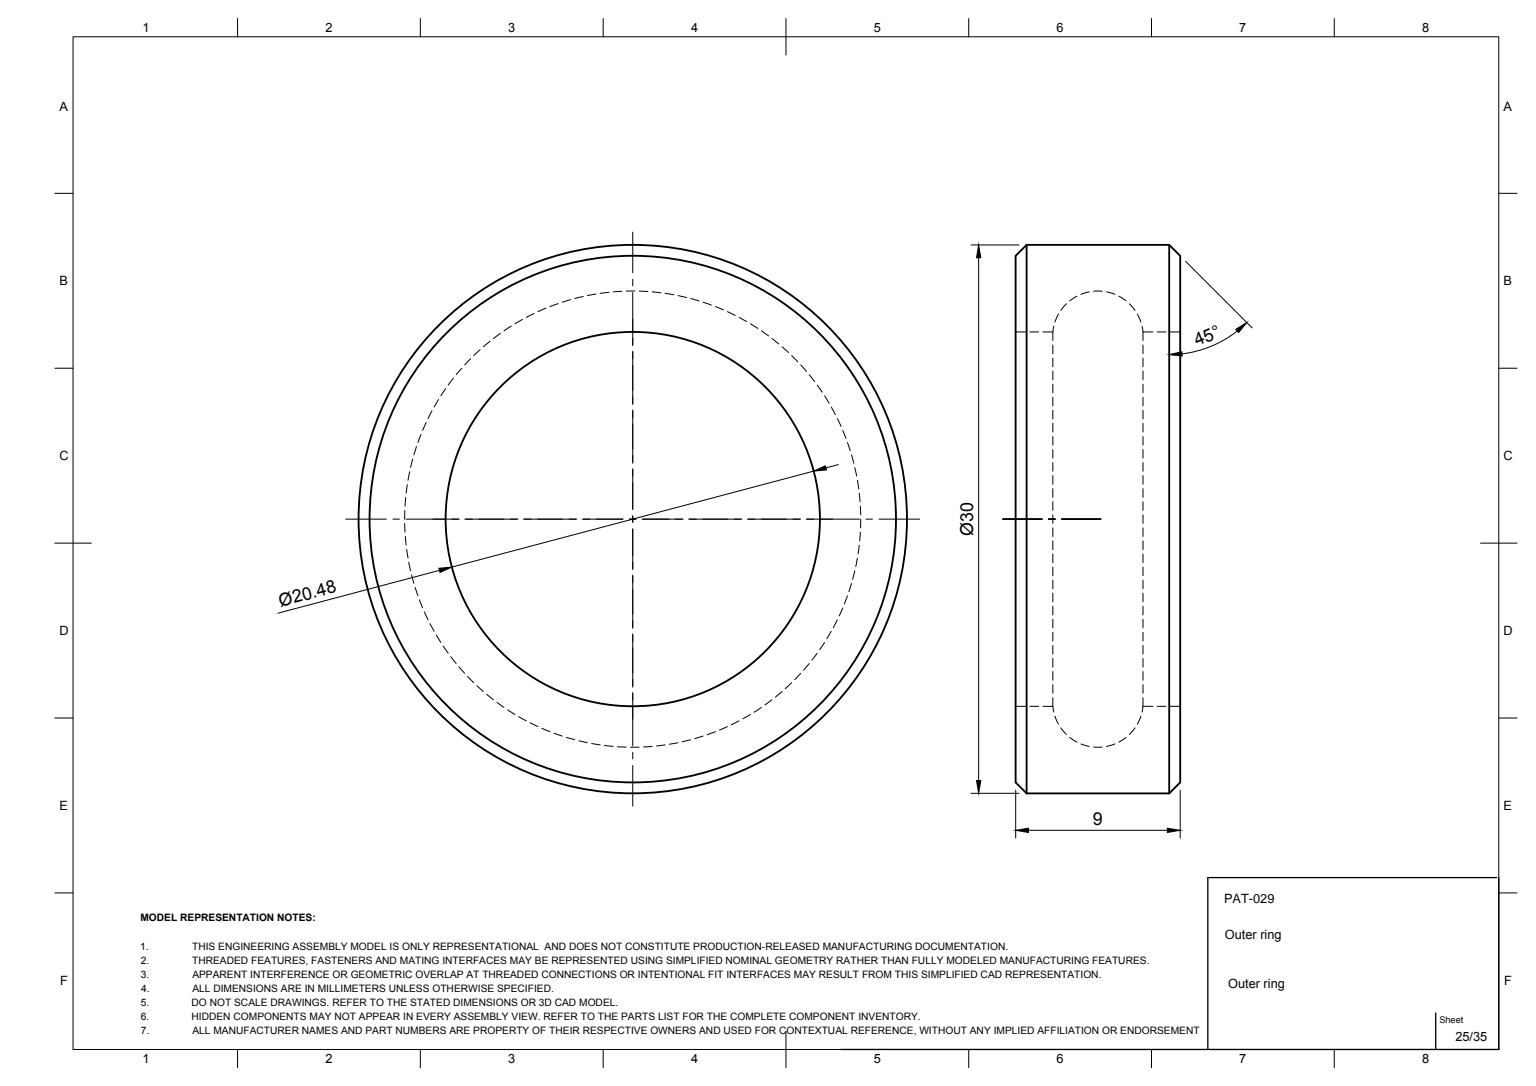
ISO-10303-21;
HEADER;
/* Generated by software containing ST-Developer
 * from STEP Tools, Inc. (www.steptools.com) 
 */

FILE_DESCRIPTION(
/* description */ ('Door-style hinge test fixture with detent'),
/* implementation_level */ '2;1');

FILE_NAME(
/* name */ 'Outer ring.step',
/* time_stamp */ '2026-10-28T03:24:57-07:00',
/* author */ (''),
/* organization */ (''),
/* preprocessor_version */ 'ST-DEVELOPER v20.2',
/* originating_system */ 'Autodesk Translation Framework v15.17.0.0',
/* authorisation */ '');

FILE_SCHEMA (('AUTOMOTIVE_DESIGN { 1 0 10303 214 3 1 1 }'));
ENDSEC;

DATA;
#10=MECHANICAL_DESIGN_GEOMETRIC_PRESENTATION_REPRESENTATION('',(#343),#9813);
#200=TOROIDAL_SURFACE('',#5464,1.,0.247676);
#206=CONICAL_SURFACE('',#5475,1.47,0.785398163397449);
#207=CONICAL_SURFACE('',#5479,1.47,0.785398163397449);
#280=SHAPE_REPRESENTATION_RELATIONSHIP('SRR','None',#9958,#311);
#311=ADVANCED_BREP_SHAPE_REPRESENTATION('',(#382),#9801);
#343=STYLED_ITEM('',(#10183),#382);
#382=MANIFOLD_SOLID_BREP('Body1',#4775);
#470=FACE_BOUND('',#1192,.T.);
#471=FACE_BOUND('',#1197,.T.);
#607=PLANE('',#5472);
#608=PLANE('',#5481);
#833=FACE_OUTER_BOUND('',#1189,.T.);
#834=FACE_OUTER_BOUND('',#1190,.T.);
#835=FACE_OUTER_BOUND('',#1191,.T.);
#836=FACE_OUTER_BOUND('',#1193,.T.);
#837=FACE_OUTER_BOUND('',#1194,.T.);
#838=FACE_OUTER_BOUND('',#1195,.T.);
#839=FACE_OUTER_BOUND('',#1196,.T.);
#840=FACE_OUTER_BOUND('',#1198,.T.);
#1189=EDGE_LOOP('',(#3931,#3932,#3933,#3934,#3935,#3936));
#1190=EDGE_LOOP('',(#3937,#3938,#3939,#3940,#3941));
#1191=EDGE_LOOP('',(#3942));
#1192=EDGE_LOOP('',(#3943));
#1193=EDGE_LOOP('',(#3944,#3945,#3946,#3947));
#1194=EDGE_LOOP('',(#3948,#3949,#3950,#3951));
#1195=EDGE_LOOP('',(#3952,#3953,#3954,#3955));
#1196=EDGE_LOOP('',(#3956));
#1197=EDGE_LOOP('',(#3957));
#1198=EDGE_LOOP('',(#3958,#3959,#3960,#3961,#3962));
#1562=LINE('',#8820,#1882);
#1563=LINE('',#8829,#1883);
#1564=LINE('',#8833,#1884);
#1565=LINE('',#8837,#1885);
#1566=LINE('',#8840,#1886);
#1882=VECTOR('',#6647,1.023815);
#1883=VECTOR('',#6658,1.47);
#1884=VECTOR('',#6663,1.5);
#1885=VECTOR('',#6668,1.47);
#1886=VECTOR('',#6673,1.023815);
#2107=CIRCLE('',#5465,1.023815);
#2108=CIRCLE('',#5466,1.023815);
#2109=CIRCLE('',#5467,0.247676);
#2110=CIRCLE('',#5468,1.023815);
#2111=CIRCLE('',#5469,1.023815);
#2112=CIRCLE('',#5471,1.023815);
#2113=CIRCLE('',#5473,1.44);
#2114=CIRCLE('',#5474,1.023815);
#2115=CIRCLE('',#5476,1.5);
#2116=CIRCLE('',#5478,1.5);
#2117=CIRCLE('',#5480,1.44);
#2462=VERTEX_POINT('',#8808);
#2463=VERTEX_POINT('',#8809);
#2464=VERTEX_POINT('',#8812);
#2465=VERTEX_POINT('',#8814);
#2466=VERTEX_POINT('',#8818);
#2467=VERTEX_POINT('',#8822);
#2468=VERTEX_POINT('',#8824);
#2469=VERTEX_POINT('',#8827);
#2470=VERTEX_POINT('',#8831);
#2471=VERTEX_POINT('',#8835);
#2982=EDGE_CURVE('',#2462,#2463,#2107,.T.);
#2983=EDGE_CURVE('',#2463,#2462,#2108,.T.);
#2984=EDGE_CURVE('',#2463,#2464,#2109,.T.);
#2985=EDGE_CURVE('',#2465,#2464,#2110,.T.);
#2986=EDGE_CURVE('',#2464,#2465,#2111,.T.);
#2987=EDGE_CURVE('',#2466,#2466,#2112,.T.);
#2988=EDGE_CURVE('',#2466,#2465,#1562,.T.);
#2989=EDGE_CURVE('',#2467,#2467,#2113,.T.);
#2990=EDGE_CURVE('',#2468,#2468,#2114,.T.);
#2991=EDGE_CURVE('',#2469,#2469,#2115,.T.);
#2992=EDGE_CURVE('',#2469,#2467,#1563,.T.);
#2993=EDGE_CURVE('',#2470,#2470,#2116,.T.);
#2994=EDGE_CURVE('',#2470,#2469,#1564,.T.);
#2995=EDGE_CURVE('',#2471,#2471,#2117,.T.);
#2996=EDGE_CURVE('',#2471,#2470,#1565,.T.);
#2997=EDGE_CURVE('',#2462,#2468,#1566,.T.);
#3931=ORIENTED_EDGE('',*,*,#2982,.F.);
#3932=ORIENTED_EDGE('',*,*,#2983,.F.);
#3933=ORIENTED_EDGE('',*,*,#2984,.T.);
#3934=ORIENTED_EDGE('',*,*,#2985,.F.);
#3935=ORIENTED_EDGE('',*,*,#2986,.F.);
#3936=ORIENTED_EDGE('',*,*,#2984,.F.);
#3937=ORIENTED_EDGE('',*,*,#2987,.T.);
#3938=ORIENTED_EDGE('',*,*,#2988,.T.);
#3939=ORIENTED_EDGE('',*,*,#2985,.T.);
#3940=ORIENTED_EDGE('',*,*,#2986,.T.);
#3941=ORIENTED_EDGE('',*,*,#2988,.F.);
#3942=ORIENTED_EDGE('',*,*,#2989,.F.);
#3943=ORIENTED_EDGE('',*,*,#2990,.T.);
#3944=ORIENTED_EDGE('',*,*,#2991,.F.);
#3945=ORIENTED_EDGE('',*,*,#2992,.T.);
#3946=ORIENTED_EDGE('',*,*,#2989,.T.);
#3947=ORIENTED_EDGE('',*,*,#2992,.F.);
#3948=ORIENTED_EDGE('',*,*,#2993,.F.);
#3949=ORIENTED_EDGE('',*,*,#2994,.T.);
#3950=ORIENTED_EDGE('',*,*,#2991,.T.);
#3951=ORIENTED_EDGE('',*,*,#2994,.F.);
#3952=ORIENTED_EDGE('',*,*,#2995,.F.);
#3953=ORIENTED_EDGE('',*,*,#2996,.T.);
#3954=ORIENTED_EDGE('',*,*,#2993,.T.);
#3955=ORIENTED_EDGE('',*,*,#2996,.F.);
#3956=ORIENTED_EDGE('',*,*,#2995,.T.);
#3957=ORIENTED_EDGE('',*,*,#2987,.F.);
#3958=ORIENTED_EDGE('',*,*,#2982,.T.);
#3959=ORIENTED_EDGE('',*,*,#2983,.T.);
#3960=ORIENTED_EDGE('',*,*,#2997,.T.);
#3961=ORIENTED_EDGE('',*,*,#2990,.F.);
#3962=ORIENTED_EDGE('',*,*,#2997,.F.);
#4436=CYLINDRICAL_SURFACE('',#5470,1.023815);
#4437=CYLINDRICAL_SURFACE('',#5477,1.5);
#4438=CYLINDRICAL_SURFACE('',#5482,1.023815);
#4638=ADVANCED_FACE('',(#833),#200,.F.);
#4639=ADVANCED_FACE('',(#834),#4436,.F.);
#4640=ADVANCED_FACE('',(#835,#470),#607,.T.);
#4641=ADVANCED_FACE('',(#836),#206,.T.);
#4642=ADVANCED_FACE('',(#837),#4437,.T.);
#4643=ADVANCED_FACE('',(#838),#207,.T.);
#4644=ADVANCED_FACE('',(#839,#471),#608,.T.);
#4645=ADVANCED_FACE('',(#840),#4438,.F.);
#4775=CLOSED_SHELL('',(#4638,#4639,#4640,#4641,#4642,#4643,#4644,#4645));
#5463=AXIS2_PLACEMENT_3D('',#8806,#6629,#6630);
#5464=AXIS2_PLACEMENT_3D('',#8807,#6631,#6632);
#5465=AXIS2_PLACEMENT_3D('',#8810,#6633,#6634);
#5466=AXIS2_PLACEMENT_3D('',#8811,#6635,#6636);
#5467=AXIS2_PLACEMENT_3D('',#8813,#6637,#6638);
#5468=AXIS2_PLACEMENT_3D('',#8815,#6639,#6640);
#5469=AXIS2_PLACEMENT_3D('',#8816,#6641,#6642);
#5470=AXIS2_PLACEMENT_3D('',#8817,#6643,#6644);
#5471=AXIS2_PLACEMENT_3D('',#8819,#6645,#6646);
#5472=AXIS2_PLACEMENT_3D('',#8821,#6648,#6649);
#5473=AXIS2_PLACEMENT_3D('',#8823,#6650,#6651);
#5474=AXIS2_PLACEMENT_3D('',#8825,#6652,#6653);
#5475=AXIS2_PLACEMENT_3D('',#8826,#6654,#6655);
#5476=AXIS2_PLACEMENT_3D('',#8828,#6656,#6657);
#5477=AXIS2_PLACEMENT_3D('',#8830,#6659,#6660);
#5478=AXIS2_PLACEMENT_3D('',#8832,#6661,#6662);
#5479=AXIS2_PLACEMENT_3D('',#8834,#6664,#6665);
#5480=AXIS2_PLACEMENT_3D('',#8836,#6666,#6667);
#5481=AXIS2_PLACEMENT_3D('',#8838,#6669,#6670);
#5482=AXIS2_PLACEMENT_3D('',#8839,#6671,#6672);
#6629=DIRECTION('axis',(0.,0.,1.));
#6630=DIRECTION('refdir',(1.,0.,0.));
#6631=DIRECTION('center_axis',(0.,-1.,0.));
#6632=DIRECTION('ref_axis',(0.,0.,-1.));
#6633=DIRECTION('center_axis',(0.,-1.,0.));
#6634=DIRECTION('ref_axis',(1.,0.,0.));
#6635=DIRECTION('center_axis',(0.,-1.,0.));
#6636=DIRECTION('ref_axis',(1.,0.,0.));
#6637=DIRECTION('center_axis',(1.,0.,1.22464679914735E-16));
#6638=DIRECTION('ref_axis',(-1.22464679914735E-16,0.,1.));
#6639=DIRECTION('center_axis',(0.,1.,0.));
#6640=DIRECTION('ref_axis',(1.,0.,0.));
#6641=DIRECTION('center_axis',(0.,1.,0.));
#6642=DIRECTION('ref_axis',(1.,0.,0.));
#6643=DIRECTION('center_axis',(0.,-1.,0.));
#6644=DIRECTION('ref_axis',(1.,0.,0.));
#6645=DIRECTION('center_axis',(0.,-1.,0.));
#6646=DIRECTION('ref_axis',(1.,0.,0.));
#6647=DIRECTION('',(0.,1.,0.));
#6648=DIRECTION('center_axis',(0.,1.,0.));
#6649=DIRECTION('ref_axis',(0.,0.,1.));
#6650=DIRECTION('center_axis',(0.,-1.,0.));
#6651=DIRECTION('ref_axis',(1.,0.,0.));
#6652=DIRECTION('center_axis',(0.,-1.,0.));
#6653=DIRECTION('ref_axis',(1.,0.,0.));
#6654=DIRECTION('center_axis',(0.,-1.,0.));
#6655=DIRECTION('ref_axis',(1.,0.,0.));
#6656=DIRECTION('center_axis',(0.,-1.,0.));
#6657=DIRECTION('ref_axis',(1.,0.,0.));
#6658=DIRECTION('',(0.707106781186548,0.707106781186547,8.65956056235494E-17));
#6659=DIRECTION('center_axis',(0.,-1.,0.));
#6660=DIRECTION('ref_axis',(1.,0.,0.));
#6661=DIRECTION('center_axis',(0.,-1.,0.));
#6662=DIRECTION('ref_axis',(1.,0.,0.));
#6663=DIRECTION('',(0.,1.,0.));
#6664=DIRECTION('center_axis',(0.,1.,0.));
#6665=DIRECTION('ref_axis',(1.,0.,0.));
#6666=DIRECTION('center_axis',(0.,-1.,0.));
#6667=DIRECTION('ref_axis',(1.,0.,0.));
#6668=DIRECTION('',(-0.707106781186548,0.707106781186547,-8.65956056235494E-17));
#6669=DIRECTION('center_axis',(0.,-1.,0.));
#6670=DIRECTION('ref_axis',(0.,0.,-1.));
#6671=DIRECTION('center_axis',(0.,-1.,0.));
#6672=DIRECTION('ref_axis',(1.,0.,0.));
#6673=DIRECTION('',(0.,1.,0.));
#8806=CARTESIAN_POINT('',(0.,0.,0.));
#8807=CARTESIAN_POINT('Origin',(0.,0.,0.));
#8808=CARTESIAN_POINT('',(-1.023815,0.246528389340863,-1.25381176266905E-16));
#8809=CARTESIAN_POINT('',(-1.25381176266905E-16,0.246528389340863,1.023815));
#8810=CARTESIAN_POINT('Origin',(0.,0.246528389340863,0.));
#8811=CARTESIAN_POINT('Origin',(0.,0.246528389340863,0.));
#8812=CARTESIAN_POINT('',(-1.25381176266905E-16,-0.246528389340863,1.023815));
#8813=CARTESIAN_POINT('Origin',(-1.22464679914735E-16,0.,1.));
#8814=CARTESIAN_POINT('',(-1.023815,-0.246528389340863,1.25381176266905E-16));
#8815=CARTESIAN_POINT('Origin',(0.,-0.246528389340863,0.));
#8816=CARTESIAN_POINT('Origin',(0.,-0.246528389340863,0.));
#8817=CARTESIAN_POINT('Origin',(0.,0.,0.));
#8818=CARTESIAN_POINT('',(-1.023815,-0.45,-1.25381176266905E-16));
#8819=CARTESIAN_POINT('Origin',(0.,-0.45,0.));
#8820=CARTESIAN_POINT('',(-1.023815,0.,-1.25381176266905E-16));
#8821=CARTESIAN_POINT('Origin',(1.44,0.45,0.));
#8822=CARTESIAN_POINT('',(-1.44,0.45,-1.76349139077219E-16));
#8823=CARTESIAN_POINT('Origin',(0.,0.45,0.));
#8824=CARTESIAN_POINT('',(-1.023815,0.45,-1.25381176266905E-16));
#8825=CARTESIAN_POINT('Origin',(0.,0.45,0.));
#8826=CARTESIAN_POINT('Origin',(0.,0.42,0.));
#8827=CARTESIAN_POINT('',(-1.5,0.39,-1.83697019872103E-16));
#8828=CARTESIAN_POINT('Origin',(0.,0.39,0.));
#8829=CARTESIAN_POINT('',(-1.47,0.42,-1.80023079474661E-16));
#8830=CARTESIAN_POINT('Origin',(0.,0.,0.));
#8831=CARTESIAN_POINT('',(-1.5,-0.39,-1.83697019872103E-16));
#8832=CARTESIAN_POINT('Origin',(0.,-0.39,0.));
#8833=CARTESIAN_POINT('',(-1.5,0.,-1.83697019872103E-16));
#8834=CARTESIAN_POINT('Origin',(0.,-0.42,0.));
#8835=CARTESIAN_POINT('',(-1.44,-0.45,-1.76349139077219E-16));
#8836=CARTESIAN_POINT('Origin',(0.,-0.45,0.));
#8837=CARTESIAN_POINT('',(-1.47,-0.42,-1.80023079474661E-16));
#8838=CARTESIAN_POINT('Origin',(1.023815,-0.45,0.));
#8839=CARTESIAN_POINT('Origin',(0.,0.,0.));
#8840=CARTESIAN_POINT('',(-1.023815,0.,-1.25381176266905E-16));
#9765=UNCERTAINTY_MEASURE_WITH_UNIT(LENGTH_MEASURE(0.001),#9814,
'DISTANCE_ACCURACY_VALUE',
'Maximum model space distance between geometric entities at asserted c
onnectivities');
#9777=UNCERTAINTY_MEASURE_WITH_UNIT(LENGTH_MEASURE(0.001),#9814,
'DISTANCE_ACCURACY_VALUE',
'Maximum model space distance between geometric entities at asserted c
onnectivities');
#9801=(
GEOMETRIC_REPRESENTATION_CONTEXT(3)
GLOBAL_UNCERTAINTY_ASSIGNED_CONTEXT((#9765))
GLOBAL_UNIT_ASSIGNED_CONTEXT((#9814,#9816,#9817))
REPRESENTATION_CONTEXT('','3D')
);
#9813=(
GEOMETRIC_REPRESENTATION_CONTEXT(3)
GLOBAL_UNCERTAINTY_ASSIGNED_CONTEXT((#9777))
GLOBAL_UNIT_ASSIGNED_CONTEXT((#9814,#9816,#9817))
REPRESENTATION_CONTEXT('','3D')
);
#9814=(
LENGTH_UNIT()
NAMED_UNIT(*)
SI_UNIT(.CENTI.,.METRE.)
);
#9816=(
NAMED_UNIT(*)
PLANE_ANGLE_UNIT()
SI_UNIT($,.RADIAN.)
);
#9817=(
NAMED_UNIT(*)
SI_UNIT($,.STERADIAN.)
SOLID_ANGLE_UNIT()
);
#9841=SHAPE_DEFINITION_REPRESENTATION(#9876,#9958);
#9876=PRODUCT_DEFINITION_SHAPE('',$,#9994);
#9958=SHAPE_REPRESENTATION('',(#5463),#9801);
#9970=PRODUCT_DEFINITION_CONTEXT('part definition',#10077,'design');
#9994=PRODUCT_DEFINITION('Outer ring','Outer ring',#10029,#9970);
#10029=PRODUCT_DEFINITION_FORMATION('',$,#10102);
#10077=APPLICATION_CONTEXT(
'Core Data for Automotive Mechanical Design Process');
#10078=PRODUCT_CONTEXT('part definition',#10077,'mechanical');
#10102=PRODUCT('Outer ring','Outer ring','Outer ring',(#10078));
#10177=COLOUR_RGB('Grey',0.48,0.52,0.57);
#10178=FILL_AREA_STYLE_COLOUR('',#10177);
#10179=FILL_AREA_STYLE('',(#10178));
#10180=SURFACE_STYLE_FILL_AREA(#10179);
#10181=SURFACE_SIDE_STYLE('',(#10180));
#10182=SURFACE_STYLE_USAGE(.BOTH.,#10181);
#10183=PRESENTATION_STYLE_ASSIGNMENT((#10182));
ENDSEC;
END-ISO-10303-21;
